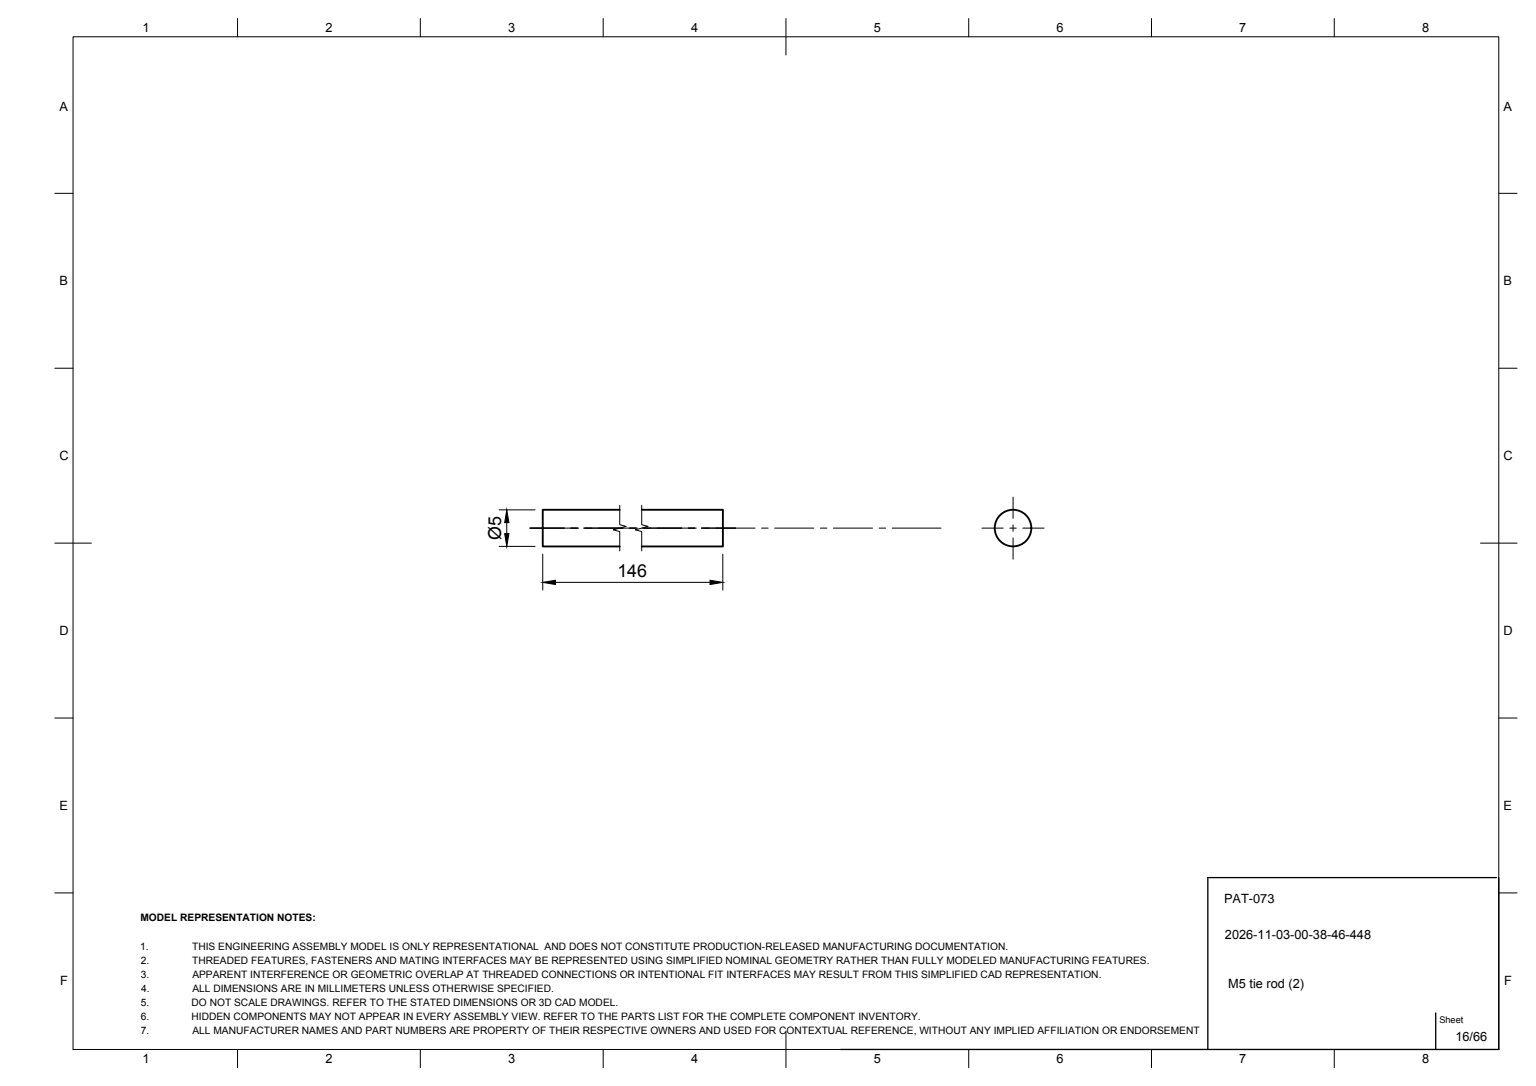
ISO-10303-21;
HEADER;
/* Generated by software containing ST-Developer
 * from STEP Tools, Inc. (www.steptools.com) 
 */

FILE_DESCRIPTION(
/* description */ ('Manual piston pump'),
/* implementation_level */ '2;1');

FILE_NAME(
/* name */ 'M5 tie rod (2).step',
/* time_stamp */ '2026-11-02T16:54:23-08:00',
/* author */ (''),
/* organization */ (''),
/* preprocessor_version */ 'ST-DEVELOPER v20.2',
/* originating_system */ 'Autodesk Translation Framework v15.17.0.0',
/* authorisation */ '');

FILE_SCHEMA (('AUTOMOTIVE_DESIGN { 1 0 10303 214 3 1 1 }'));
ENDSEC;

DATA;
#10=MECHANICAL_DESIGN_GEOMETRIC_PRESENTATION_REPRESENTATION('',(#699),#19043);
#573=SHAPE_REPRESENTATION_RELATIONSHIP('SRR','None',#19319,#636);
#636=ADVANCED_BREP_SHAPE_REPRESENTATION('',(#771),#18986);
#699=STYLED_ITEM('',(#19661),#771);
#771=MANIFOLD_SOLID_BREP('Body1',#9483);
#1140=CYLINDRICAL_SURFACE('',#10466,0.25);
#1399=FACE_OUTER_BOUND('',#2031,.T.);
#1400=FACE_OUTER_BOUND('',#2032,.T.);
#1401=FACE_OUTER_BOUND('',#2033,.T.);
#2031=EDGE_LOOP('',(#6723,#6724,#6725,#6726));
#2032=EDGE_LOOP('',(#6727));
#2033=EDGE_LOOP('',(#6728));
#2765=CIRCLE('',#10467,0.25);
#2766=CIRCLE('',#10468,0.25);
#3267=LINE('',#15153,#3871);
#3871=VECTOR('',#12065,0.25);
#4504=VERTEX_POINT('',#15150);
#4505=VERTEX_POINT('',#15152);
#5348=EDGE_CURVE('',#4504,#4504,#2765,.T.);
#5349=EDGE_CURVE('',#4504,#4505,#3267,.T.);
#5350=EDGE_CURVE('',#4505,#4505,#2766,.T.);
#6723=ORIENTED_EDGE('',*,*,#5348,.F.);
#6724=ORIENTED_EDGE('',*,*,#5349,.T.);
#6725=ORIENTED_EDGE('',*,*,#5350,.T.);
#6726=ORIENTED_EDGE('',*,*,#5349,.F.);
#6727=ORIENTED_EDGE('',*,*,#5348,.T.);
#6728=ORIENTED_EDGE('',*,*,#5350,.F.);
#8630=PLANE('',#10469);
#8631=PLANE('',#10470);
#9004=ADVANCED_FACE('',(#1399),#1140,.T.);
#9005=ADVANCED_FACE('',(#1400),#8630,.T.);
#9006=ADVANCED_FACE('',(#1401),#8631,.F.);
#9483=CLOSED_SHELL('',(#9004,#9005,#9006));
#10465=AXIS2_PLACEMENT_3D('',#15148,#12059,#12060);
#10466=AXIS2_PLACEMENT_3D('',#15149,#12061,#12062);
#10467=AXIS2_PLACEMENT_3D('',#15151,#12063,#12064);
#10468=AXIS2_PLACEMENT_3D('',#15154,#12066,#12067);
#10469=AXIS2_PLACEMENT_3D('',#15155,#12068,#12069);
#10470=AXIS2_PLACEMENT_3D('',#15156,#12070,#12071);
#12059=DIRECTION('axis',(0.,0.,1.));
#12060=DIRECTION('refdir',(1.,0.,0.));
#12061=DIRECTION('center_axis',(0.,1.,0.));
#12062=DIRECTION('ref_axis',(1.,0.,0.));
#12063=DIRECTION('center_axis',(0.,1.,0.));
#12064=DIRECTION('ref_axis',(1.,0.,0.));
#12065=DIRECTION('',(0.,-1.,0.));
#12066=DIRECTION('center_axis',(0.,1.,0.));
#12067=DIRECTION('ref_axis',(1.,0.,0.));
#12068=DIRECTION('center_axis',(0.,1.,0.));
#12069=DIRECTION('ref_axis',(1.,0.,0.));
#12070=DIRECTION('center_axis',(0.,1.,0.));
#12071=DIRECTION('ref_axis',(1.,0.,0.));
#15148=CARTESIAN_POINT('',(0.,0.,0.));
#15149=CARTESIAN_POINT('Origin',(2.,-1.,2.5));
#15150=CARTESIAN_POINT('',(1.75,13.6,2.5));
#15151=CARTESIAN_POINT('Origin',(2.,13.6,2.5));
#15152=CARTESIAN_POINT('',(1.75,-1.,2.5));
#15153=CARTESIAN_POINT('',(1.75,-1.,2.5));
#15154=CARTESIAN_POINT('Origin',(2.,-1.,2.5));
#15155=CARTESIAN_POINT('Origin',(2.,13.6,2.5));
#15156=CARTESIAN_POINT('Origin',(2.,-1.,2.5));
#18915=UNCERTAINTY_MEASURE_WITH_UNIT(LENGTH_MEASURE(0.001),#19044,
'DISTANCE_ACCURACY_VALUE',
'Maximum model space distance between geometric entities at asserted c
onnectivities');
#18972=UNCERTAINTY_MEASURE_WITH_UNIT(LENGTH_MEASURE(0.001),#19044,
'DISTANCE_ACCURACY_VALUE',
'Maximum model space distance between geometric entities at asserted c
onnectivities');
#18986=(
GEOMETRIC_REPRESENTATION_CONTEXT(3)
GLOBAL_UNCERTAINTY_ASSIGNED_CONTEXT((#18915))
GLOBAL_UNIT_ASSIGNED_CONTEXT((#19044,#19046,#19047))
REPRESENTATION_CONTEXT('','3D')
);
#19043=(
GEOMETRIC_REPRESENTATION_CONTEXT(3)
GLOBAL_UNCERTAINTY_ASSIGNED_CONTEXT((#18972))
GLOBAL_UNIT_ASSIGNED_CONTEXT((#19044,#19046,#19047))
REPRESENTATION_CONTEXT('','3D')
);
#19044=(
LENGTH_UNIT()
NAMED_UNIT(*)
SI_UNIT(.CENTI.,.METRE.)
);
#19046=(
NAMED_UNIT(*)
PLANE_ANGLE_UNIT()
SI_UNIT($,.RADIAN.)
);
#19047=(
NAMED_UNIT(*)
SI_UNIT($,.STERADIAN.)
SOLID_ANGLE_UNIT()
);
#19061=SHAPE_DEFINITION_REPRESENTATION(#19131,#19319);
#19131=PRODUCT_DEFINITION_SHAPE('',$,#19390);
#19319=SHAPE_REPRESENTATION('',(#10465),#18986);
#19376=PRODUCT_DEFINITION_CONTEXT('part definition',#19588,'design');
#19390=PRODUCT_DEFINITION('2026-11-03-00-38-46-448','M5 tie rod (2)',#19460,
#19376);
#19460=PRODUCT_DEFINITION_FORMATION('',$,#19603);
#19588=APPLICATION_CONTEXT(
'Core Data for Automotive Mechanical Design Process');
#19589=PRODUCT_CONTEXT('part definition',#19588,'mechanical');
#19603=PRODUCT('2026-11-03-00-38-46-448','M5 tie rod (2)','M5 tie rod',
(#19589));
#19661=PRESENTATION_STYLE_ASSIGNMENT((#19667));
#19667=SURFACE_STYLE_USAGE(.BOTH.,#19673);
#19673=SURFACE_SIDE_STYLE('',(#19679));
#19679=SURFACE_STYLE_FILL_AREA(#19685);
#19685=FILL_AREA_STYLE('CAD Library Painted - Engineering blue',(#19691));
#19691=FILL_AREA_STYLE_COLOUR('CAD Library Painted - Engineering blue',
#19697);
#19697=COLOUR_RGB('CAD Library Painted - Engineering blue',0.12156862745098,
0.356862745098039,0.6);
ENDSEC;
END-ISO-10303-21;
